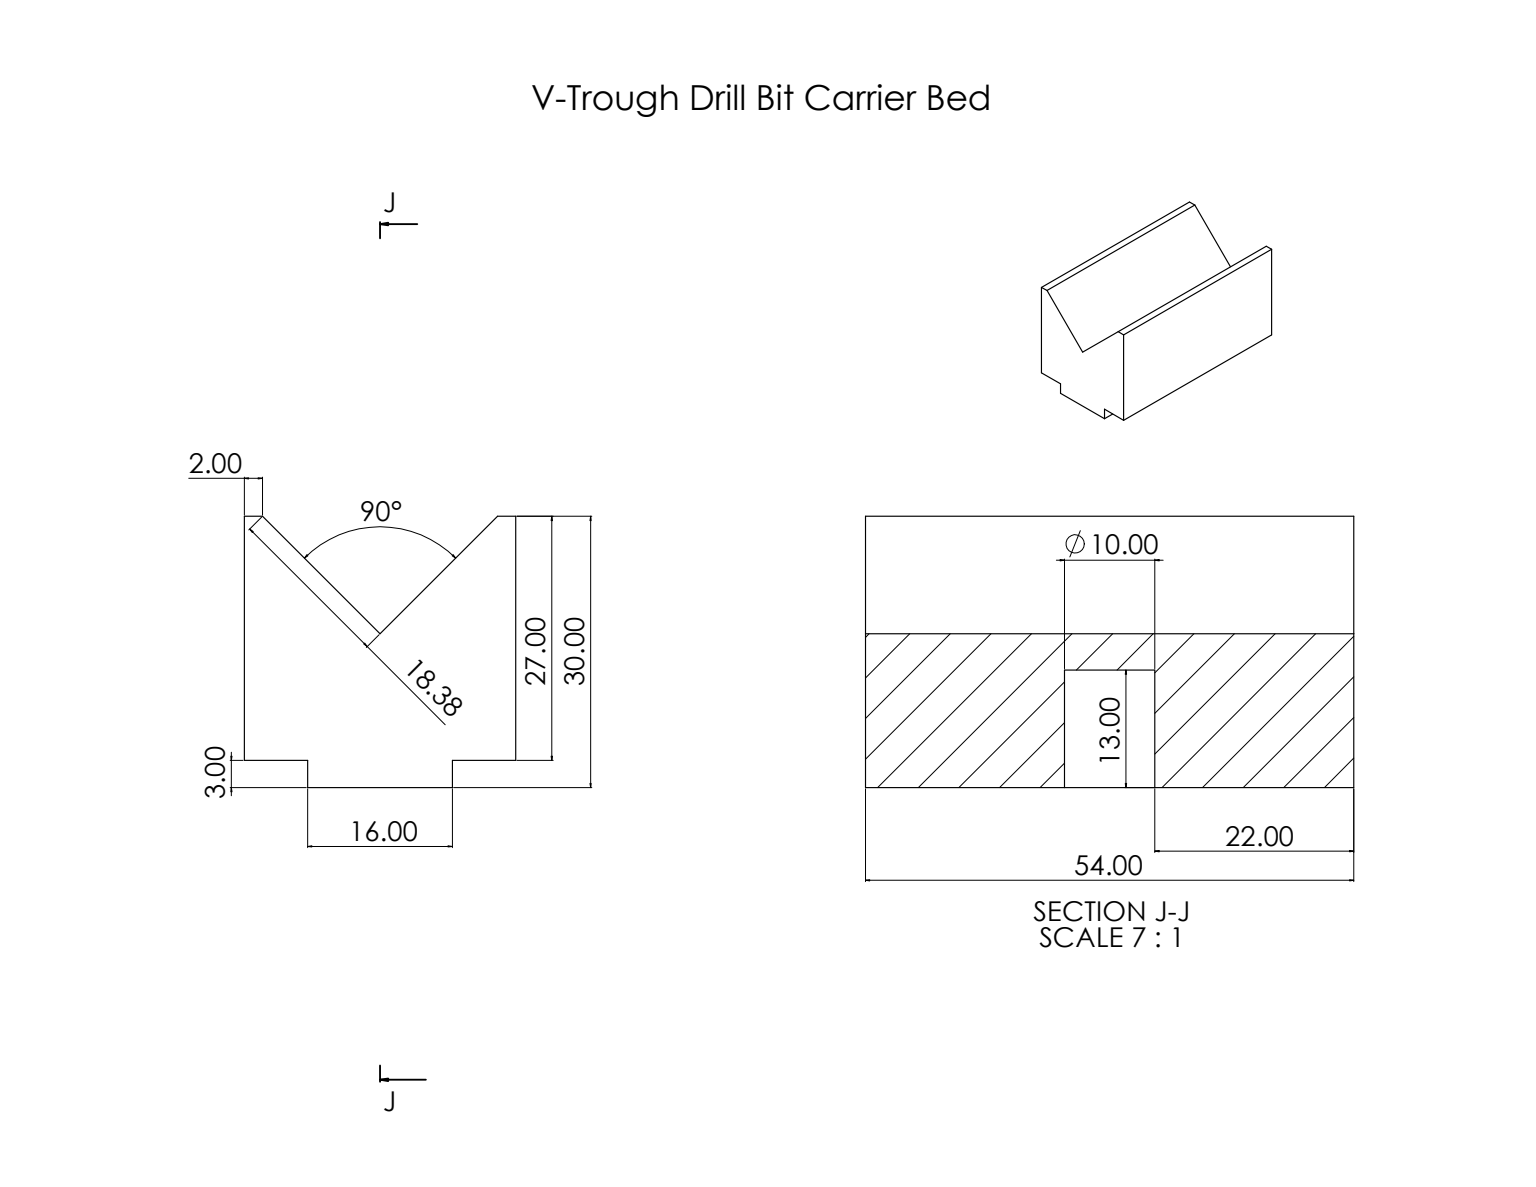
ISO-10303-21;
HEADER;
FILE_DESCRIPTION (('STEP AP214'),
    '1' );
FILE_NAME ('V-Trough Drill Bit Carrier Bed.step',
    '2026-10-26T22:46:44',
    ( '' ),
    ( '' ),
    'SwSTEP 2.0',
    'SolidWorks 2025',
    '' );
FILE_SCHEMA (( 'AUTOMOTIVE_DESIGN' ));
ENDSEC;

DATA;
#6=ORIENTED_EDGE ( 'NONE', *, *, #8024, .T. ) ;
#20=LINE ( 'NONE', #125, #6600 ) ;
#91=EDGE_CURVE ( 'NONE', #17637, #19670, #15056, .T. ) ;
#99=ORIENTED_EDGE ( 'NONE', *, *, #8969, .F. ) ;
#125=CARTESIAN_POINT ( 'NONE',  ( 74.11964624731606932, 223.5773763115391262, -13.99999999999998757 ) ) ;
#138=VECTOR ( 'NONE', #4761, 1000.000000000000114 ) ;
#144=ORIENTED_EDGE ( 'NONE', *, *, #2804, .F. ) ;
#147=CARTESIAN_POINT ( 'NONE',  ( 59.39721438298058587, 215.0773763115390125, -5.999999999999973355 ) ) ;
#214=ORIENTED_EDGE ( 'NONE', *, *, #1106, .F. ) ;
#252=ORIENTED_EDGE ( 'NONE', *, *, #4604, .T. ) ;
#276=DIRECTION ( 'NONE',  ( 0.000000000000000000, 0.000000000000000000, -1.000000000000000000 ) ) ;
#283=DIRECTION ( 'NONE',  ( -0.8660254037844370423, -0.5000000000000027756, 0.000000000000000000 ) ) ;
#292=ORIENTED_EDGE ( 'NONE', *, *, #18582, .T. ) ;
#382=AXIS2_PLACEMENT_3D ( 'NONE', #19245, #4714, #11186 ) ;
#397=DIRECTION ( 'NONE',  ( -0.8660254037844360431, -0.5000000000000046629, 0.000000000000000000 ) ) ;
#416=LINE ( 'NONE', #6862, #13294 ) ;
#757=DIRECTION ( 'NONE',  ( -3.965082230804136925E-15, -7.930164461608273850E-15, 1.000000000000000000 ) ) ;
#780=CARTESIAN_POINT ( 'NONE',  ( 61.99529059433385925, 216.5773763115390125, -5.999999999999973355 ) ) ;
#823=EDGE_LOOP ( 'NONE', ( #9472, #292, #20590, #17271 ) ) ;
#881=PLANE ( 'NONE',  #5818 ) ;
#968=EDGE_CURVE ( 'NONE', #15204, #2259, #12531, .T. ) ;
#983=CIRCLE ( 'NONE', #5694, 5.000000000000005329 ) ;
#986=PRODUCT_DEFINITION_FORMATION_WITH_SPECIFIED_SOURCE ( 'ANY', '', #7367, .NOT_KNOWN. ) ;
#1094=( GEOMETRIC_REPRESENTATION_CONTEXT ( 3 ) GLOBAL_UNCERTAINTY_ASSIGNED_CONTEXT ( ( #5747 ) ) GLOBAL_UNIT_ASSIGNED_CONTEXT ( ( #17535, #19424, #17849 ) ) REPRESENTATION_CONTEXT ( 'NONE', 'WORKASPACE' ) );
#1106=EDGE_CURVE ( 'NONE', #19041, #17375, #6452, .T. ) ;
#1124=LINE ( 'NONE', #12466, #4797 ) ;
#1130=DIRECTION ( 'NONE',  ( -0.8660254037844370423, -0.5000000000000027756, -0.000000000000000000 ) ) ;
#1156=VECTOR ( 'NONE', #15622, 1000.000000000000000 ) ;
#1183=ORIENTED_EDGE ( 'NONE', *, *, #12632, .F. ) ;
#1214=VECTOR ( 'NONE', #5254, 1000.000000000000227 ) ;
#1274=DIRECTION ( 'NONE',  ( 0.000000000000000000, 0.000000000000000000, 1.000000000000000000 ) ) ;
#1588=VERTEX_POINT ( 'NONE', #19080 ) ;
#1594=VERTEX_POINT ( 'NONE', #18972 ) ;
#1643=ORIENTED_EDGE ( 'NONE', *, *, #12632, .T. ) ;
#1738=DIRECTION ( 'NONE',  ( -3.965082230804136925E-15, -7.930164461608273850E-15, 1.000000000000000000 ) ) ;
#1796=SHAPE_REPRESENTATION ( 'V-Trough Drill Bit Carrier Bed', ( #18233 ), #14188 ) ;
#1868=ORIENTED_EDGE ( 'NONE', *, *, #14937, .T. ) ;
#1885=DIRECTION ( 'NONE',  ( 0.8660254037844348218, 0.5000000000000064393, 0.000000000000000000 ) ) ;
#1887=DIRECTION ( 'NONE',  ( -0.5000000000000045519, 0.8660254037844360431, 0.000000000000000000 ) ) ;
#1915=EDGE_LOOP ( 'NONE', ( #17865, #19620, #6, #15097 ) ) ;
#1955=AXIS2_PLACEMENT_3D ( 'NONE', #14799, #5313, #4911 ) ;
#1958=VERTEX_POINT ( 'NONE', #20807 ) ;
#2005=ADVANCED_FACE ( 'NONE', ( #9459 ), #4907, .F. ) ;
#2016=VERTEX_POINT ( 'NONE', #6380 ) ;
#2098=VERTEX_POINT ( 'NONE', #9771 ) ;
#2104=EDGE_LOOP ( 'NONE', ( #1183, #10709, #4662, #6785 ) ) ;
#2110=EDGE_CURVE ( 'NONE', #2016, #10851, #18262, .T. ) ;
#2208=DIRECTION ( 'NONE',  ( -0.5000000000000045519, 0.8660254037844360431, 0.000000000000000000 ) ) ;
#2259=VERTEX_POINT ( 'NONE', #4046 ) ;
#2305=PLANE ( 'NONE',  #19993 ) ;
#2322=FACE_OUTER_BOUND ( 'NONE', #2755, .T. ) ;
#2325=VERTEX_POINT ( 'NONE', #7748 ) ;
#2343=CARTESIAN_POINT ( 'NONE',  ( 74.11964624731606932, 223.5773763115391262, -13.99999999999998757 ) ) ;
#2376=VECTOR ( 'NONE', #276, 1000.000000000000000 ) ;
#2395=LINE ( 'NONE', #5765, #14247 ) ;
#2423=ADVANCED_FACE ( 'NONE', ( #9545 ), #20784, .T. ) ;
#2503=AXIS2_PLACEMENT_3D ( 'NONE', #12544, #7650, #2794 ) ;
#2539=VERTEX_POINT ( 'NONE', #11222 ) ;
#2566=EDGE_CURVE ( 'NONE', #19041, #1588, #11424, .T. ) ;
#2697=DIRECTION ( 'NONE',  ( -0.5000000000000027756, 0.8660254037844370423, -4.885182764539217401E-15 ) ) ;
#2755=EDGE_LOOP ( 'NONE', ( #15288, #4387, #20400, #14266 ) ) ;
#2772=ADVANCED_FACE ( 'NONE', ( #10120 ), #2305, .T. ) ;
#2773=VERTEX_POINT ( 'NONE', #6735 ) ;
#2776=ORIENTED_EDGE ( 'NONE', *, *, #4882, .F. ) ;
#2794=DIRECTION ( 'NONE',  ( -0.7559289460184535070, 0.000000000000000000, -0.6546536707079781969 ) ) ;
#2804=EDGE_CURVE ( 'NONE', #9345, #7191, #6784, .T. ) ;
#2819=DIRECTION ( 'NONE',  ( 0.8660254037844370423, 0.5000000000000027756, 0.000000000000000000 ) ) ;
#2887=DIRECTION ( 'NONE',  ( -0.8660254037844362651, -0.5000000000000045519, 5.976026924694053325E-17 ) ) ;
#2949=VERTEX_POINT ( 'NONE', #17764 ) ;
#2995=DIRECTION ( 'NONE',  ( 0.5000000000000045519, -0.8660254037844360431, 0.000000000000000000 ) ) ;
#3089=EDGE_CURVE ( 'NONE', #5258, #2325, #16478, .T. ) ;
#3121=DIRECTION ( 'NONE',  ( -0.8660254037844360431, -0.5000000000000044409, 5.976026924694052093E-17 ) ) ;
#3123=CARTESIAN_POINT ( 'NONE',  ( 61.99529059433388767, 216.5773763115390693, -28.99999999999998934 ) ) ;
#3124=ORIENTED_EDGE ( 'NONE', *, *, #968, .T. ) ;
#3158=ORIENTED_EDGE ( 'NONE', *, *, #14937, .F. ) ;
#3194=DIRECTION ( 'NONE',  ( -0.8660254037844360431, -0.5000000000000045519, -7.398944170774820286E-15 ) ) ;
#3316=ORIENTED_EDGE ( 'NONE', *, *, #3433, .F. ) ;
#3331=MANIFOLD_SOLID_BREP ( 'Cut-Extrude5', #10659 ) ;
#3424=FACE_OUTER_BOUND ( 'NONE', #20462, .T. ) ;
#3426=EDGE_CURVE ( 'NONE', #17375, #2098, #9056, .T. ) ;
#3433=EDGE_CURVE ( 'NONE', #18964, #2773, #2395, .T. ) ;
#3547=ORIENTED_EDGE ( 'NONE', *, *, #13844, .T. ) ;
#3597=CARTESIAN_POINT ( 'NONE',  ( 58.37797649651341203, 276.8427481158987007, -26.99999999999999289 ) ) ;
#3605=CARTESIAN_POINT ( 'NONE',  ( 61.99529059433388767, 216.5773763115390693, 1.000000000000017097 ) ) ;
#3728=CARTESIAN_POINT ( 'NONE',  ( 85.37797649651368204, 230.0773763115391262, -26.99999999999999289 ) ) ;
#3788=CARTESIAN_POINT ( 'NONE',  ( 85.37797649651368204, 230.0773763115391262, -28.99999999999998934 ) ) ;
#3847=VECTOR ( 'NONE', #6152, 1000.000000000000114 ) ;
#3889=LINE ( 'NONE', #10341, #13471 ) ;
#3959=DIRECTION ( 'NONE',  ( -0.8660254037844370423, -0.5000000000000027756, 0.000000000000000000 ) ) ;
#3988=CARTESIAN_POINT ( 'NONE',  ( 85.37797649651368204, 230.0773763115391262, -28.99999999999998934 ) ) ;
#4046=CARTESIAN_POINT ( 'NONE',  ( 58.37797649651341203, 276.8427481158987007, -0.9999999999999826805 ) ) ;
#4155=CARTESIAN_POINT ( 'NONE',  ( 58.37797649651341203, 276.8427481158987007, 1.000000000000017097 ) ) ;
#4215=CARTESIAN_POINT ( 'NONE',  ( 85.37797649651368204, 230.0773763115391262, -26.99999999999999289 ) ) ;
#4282=EDGE_LOOP ( 'NONE', ( #144, #17540 ) ) ;
#4380=LINE ( 'NONE', #18697, #12901 ) ;
#4387=ORIENTED_EDGE ( 'NONE', *, *, #7070, .F. ) ;
#4476=LINE ( 'NONE', #18685, #13839 ) ;
#4604=EDGE_CURVE ( 'NONE', #4855, #18774, #12621, .T. ) ;
#4642=ORIENTED_EDGE ( 'NONE', *, *, #2566, .T. ) ;
#4662=ORIENTED_EDGE ( 'NONE', *, *, #11730, .T. ) ;
#4677=CARTESIAN_POINT ( 'NONE',  ( 61.99529059433388767, 216.5773763115390693, -28.99999999999998934 ) ) ;
#4714=DIRECTION ( 'NONE',  ( -0.8660254037844360431, -0.5000000000000045519, 0.000000000000000000 ) ) ;
#4754=CARTESIAN_POINT ( 'NONE',  ( 34.99529059433359635, 263.3427481158985870, -22.00000000000000355 ) ) ;
#4761=DIRECTION ( 'NONE',  ( 0.8660254037844348218, 0.5000000000000064393, 0.000000000000000000 ) ) ;
#4787=VECTOR ( 'NONE', #16383, 1000.000000000000000 ) ;
#4797=VECTOR ( 'NONE', #2819, 1000.000000000000114 ) ;
#4814=CYLINDRICAL_SURFACE ( 'NONE', #1955, 5.000000000000005329 ) ;
#4855=VERTEX_POINT ( 'NONE', #12972 ) ;
#4882=EDGE_CURVE ( 'NONE', #2539, #19041, #13377, .T. ) ;
#4907=CYLINDRICAL_SURFACE ( 'NONE', #13362, 5.000000000000005329 ) ;
#4911=DIRECTION ( 'NONE',  ( 0.5000000000000041078, -0.8660254037844363761, 0.000000000000000000 ) ) ;
#5011=DIRECTION ( 'NONE',  ( -0.5000000000000045519, 0.8660254037844360431, 0.000000000000000000 ) ) ;
#5026=CARTESIAN_POINT ( 'NONE',  ( 32.39721438298032297, 261.8427481158985870, -22.00000000000000355 ) ) ;
#5056=DIRECTION ( 'NONE',  ( 0.8660254037844360431, 0.5000000000000045519, -0.000000000000000000 ) ) ;
#5062=DIRECTION ( 'NONE',  ( 0.5000000000000044409, -0.8660254037844361541, 0.000000000000000000 ) ) ;
#5077=EDGE_LOOP ( 'NONE', ( #10295, #3158, #12362, #12866 ) ) ;
#5087=CARTESIAN_POINT ( 'NONE',  ( 43.39721438298041534, 242.7901892326410120, -13.99999999999998046 ) ) ;
#5168=VECTOR ( 'NONE', #757, 1000.000000000000000 ) ;
#5171=ORIENTED_EDGE ( 'NONE', *, *, #9282, .F. ) ;
#5254=DIRECTION ( 'NONE',  ( -0.6123724356957914727, -0.3535533905932749521, -0.7071067811865495711 ) ) ;
#5258=VERTEX_POINT ( 'NONE', #20026 ) ;
#5313=DIRECTION ( 'NONE',  ( -0.8660254037844360431, -0.5000000000000044409, 5.976026924694052093E-17 ) ) ;
#5370=DIRECTION ( 'NONE',  ( 1.000000000000000000, 0.000000000000000000, -0.000000000000000000 ) ) ;
#5433=( LENGTH_UNIT ( ) NAMED_UNIT ( * ) SI_UNIT ( .MILLI., .METRE. ) );
#5452=DIRECTION ( 'NONE',  ( -0.000000000000000000, -0.000000000000000000, -1.000000000000000000 ) ) ;
#5538=PLANE ( 'NONE',  #16869 ) ;
#5564=EDGE_CURVE ( 'NONE', #2098, #5258, #8016, .T. ) ;
#5566=DIRECTION ( 'NONE',  ( -0.8660254037844360431, -0.5000000000000045519, 7.398944170774818708E-15 ) ) ;
#5638=FACE_OUTER_BOUND ( 'NONE', #20459, .T. ) ;
#5660=DIRECTION ( 'NONE',  ( -0.8660254037844370423, -0.5000000000000027756, -0.000000000000000000 ) ) ;
#5667=CARTESIAN_POINT ( 'NONE',  ( 57.15554463217811332, 244.9600622137188850, -13.99999999999998046 ) ) ;
#5683=CARTESIAN_POINT ( 'NONE',  ( 61.99529059433388767, 216.5773763115390693, 1.000000000000017097 ) ) ;
#5694=AXIS2_PLACEMENT_3D ( 'NONE', #17303, #2887, #5938 ) ;
#5735=DIRECTION ( 'NONE',  ( 0.6123724356957914727, 0.3535533905932749521, -0.7071067811865495711 ) ) ;
#5747=UNCERTAINTY_MEASURE_WITH_UNIT (LENGTH_MEASURE( 1.000000000000000082E-05 ), #17535, 'distance_accuracy_value', 'NONE');
#5764=EDGE_CURVE ( 'NONE', #2325, #15204, #1124, .T. ) ;
#5765=CARTESIAN_POINT ( 'NONE',  ( 61.99529059433388767, 216.5773763115390693, -28.99999999999998934 ) ) ;
#5778=CARTESIAN_POINT ( 'NONE',  ( 45.89721438298043665, 238.4600622137188282, -13.99999999999998046 ) ) ;
#5811=EDGE_LOOP ( 'NONE', ( #20591, #9670, #12240, #1868 ) ) ;
#5818=AXIS2_PLACEMENT_3D ( 'NONE', #15325, #13818, #20068 ) ;
#5890=PLANE ( 'NONE',  #16334 ) ;
#5907=ADVANCED_FACE ( 'NONE', ( #11803 ), #881, .T. ) ;
#5935=PRODUCT_CONTEXT ( 'NONE', #15314, 'mechanical' ) ;
#5938=DIRECTION ( 'NONE',  ( 0.5000000000000041078, -0.8660254037844363761, 0.000000000000000000 ) ) ;
#5981=FACE_BOUND ( 'NONE', #4282, .T. ) ;
#6003=CARTESIAN_POINT ( 'NONE',  ( 85.37797649651368204, 230.0773763115391262, -28.99999999999998934 ) ) ;
#6083=PLANE ( 'NONE',  #382 ) ;
#6111=ORIENTED_EDGE ( 'NONE', *, *, #7734, .F. ) ;
#6152=DIRECTION ( 'NONE',  ( -0.5000000000000045519, 0.8660254037844360431, 0.000000000000000000 ) ) ;
#6350=VECTOR ( 'NONE', #8825, 1000.000000000000114 ) ;
#6380=CARTESIAN_POINT ( 'NONE',  ( 85.37797649651368204, 230.0773763115391262, -26.99999999999999289 ) ) ;
#6382=DIRECTION ( 'NONE',  ( 1.000000000000000000, 0.000000000000000000, -0.000000000000000000 ) ) ;
#6410=CARTESIAN_POINT ( 'NONE',  ( 85.37797649651368204, 230.0773763115391262, 1.000000000000017097 ) ) ;
#6452=LINE ( 'NONE', #17821, #3847 ) ;
#6458=CARTESIAN_POINT ( 'NONE',  ( 59.65554463217813463, 240.6299351947967011, -13.99999999999998046 ) ) ;
#6512=LINE ( 'NONE', #6616, #13600 ) ;
#6521=DIRECTION ( 'NONE',  ( 0.5000000000000041078, -0.8660254037844363761, 0.000000000000000000 ) ) ;
#6559=DIRECTION ( 'NONE',  ( -0.5000000000000045519, 0.8660254037844360431, 0.000000000000000000 ) ) ;
#6564=DIRECTION ( 'NONE',  ( -0.8660254037844361541, -0.5000000000000044409, 5.976026924694052093E-17 ) ) ;
#6600=VECTOR ( 'NONE', #6559, 1000.000000000000114 ) ;
#6616=CARTESIAN_POINT ( 'NONE',  ( 85.37797649651368204, 230.0773763115391262, -0.9999999999999826805 ) ) ;
#6636=AXIS2_PLACEMENT_3D ( 'NONE', #8437, #11527, #1887 ) ;
#6644=PLANE ( 'NONE',  #13908 ) ;
#6655=ORIENTED_EDGE ( 'NONE', *, *, #2804, .T. ) ;
#6712=ORIENTED_EDGE ( 'NONE', *, *, #3426, .T. ) ;
#6735=CARTESIAN_POINT ( 'NONE',  ( 61.99529059433388767, 216.5773763115390693, -28.99999999999998934 ) ) ;
#6784=CIRCLE ( 'NONE', #17992, 5.000000000000005329 ) ;
#6785=ORIENTED_EDGE ( 'NONE', *, *, #17239, .T. ) ;
#6862=CARTESIAN_POINT ( 'NONE',  ( 61.99529059433385925, 216.5773763115390125, -5.999999999999973355 ) ) ;
#6969=DIRECTION ( 'NONE',  ( 0.000000000000000000, 0.000000000000000000, -1.000000000000000000 ) ) ;
#6987=VECTOR ( 'NONE', #8149, 1000.000000000000227 ) ;
#6993=LINE ( 'NONE', #8591, #8467 ) ;
#7058=CARTESIAN_POINT ( 'NONE',  ( 32.39721438298032297, 261.8427481158985870, -5.999999999999973355 ) ) ;
#7070=EDGE_CURVE ( 'NONE', #1958, #2325, #6993, .T. ) ;
#7191=VERTEX_POINT ( 'NONE', #5087 ) ;
#7276=PLANE ( 'NONE',  #18043 ) ;
#7367=PRODUCT ( 'V-Trough Drill Bit Carrier Bed', 'V-Trough Drill Bit Carrier Bed', '', ( #5935 ) ) ;
#7396=CARTESIAN_POINT ( 'NONE',  ( 85.37797649651368204, 230.0773763115391262, 1.000000000000017097 ) ) ;
#7569=ADVANCED_FACE ( 'NONE', ( #10134 ), #6644, .T. ) ;
#7604=LINE ( 'NONE', #6003, #17983 ) ;
#7618=ADVANCED_FACE ( 'NONE', ( #2322 ), #7276, .T. ) ;
#7650=DIRECTION ( 'NONE',  ( 0.6123724356957944703, 0.3535533905932780607, -0.7071067811865454633 ) ) ;
#7734=EDGE_CURVE ( 'NONE', #11978, #5258, #10775, .T. ) ;
#7739=ORIENTED_EDGE ( 'NONE', *, *, #17717, .T. ) ;
#7748=CARTESIAN_POINT ( 'NONE',  ( 34.99529059433362477, 263.3427481158986438, 1.000000000000017097 ) ) ;
#7815=ADVANCED_BREP_SHAPE_REPRESENTATION ( '', ( #3331, #18233 ), #14188 ) ;
#7887=ORIENTED_EDGE ( 'NONE', *, *, #8024, .F. ) ;
#7913=ORIENTED_EDGE ( 'NONE', *, *, #10333, .F. ) ;
#7922=EDGE_LOOP ( 'NONE', ( #11863, #6111, #10020, #18675 ) ) ;
#7955=LINE ( 'NONE', #6458, #10564 ) ;
#8016=LINE ( 'NONE', #7058, #8477 ) ;
#8024=EDGE_CURVE ( 'NONE', #16809, #17637, #14825, .T. ) ;
#8111=CARTESIAN_POINT ( 'NONE',  ( 45.89721438298043665, 238.4600622137188282, -13.99999999999998046 ) ) ;
#8125=EDGE_CURVE ( 'NONE', #2949, #15199, #8853, .T. ) ;
#8149=DIRECTION ( 'NONE',  ( 0.6123724356957914727, 0.3535533905932749521, -0.7071067811865495711 ) ) ;
#8220=FACE_OUTER_BOUND ( 'NONE', #20198, .T. ) ;
#8272=CARTESIAN_POINT ( 'NONE',  ( 61.99529059433385925, 216.5773763115390125, -22.00000000000000355 ) ) ;
#8287=PLANE ( 'NONE',  #8526 ) ;
#8291=LINE ( 'NONE', #11599, #11107 ) ;
#8351=CARTESIAN_POINT ( 'NONE',  ( 61.99529059433385925, 216.5773763115390125, -22.00000000000000355 ) ) ;
#8437=CARTESIAN_POINT ( 'NONE',  ( 85.37797649651368204, 230.0773763115391262, 1.000000000000017097 ) ) ;
#8452=DIRECTION ( 'NONE',  ( -1.000000000000000000, 0.000000000000000000, 0.000000000000000000 ) ) ;
#8467=VECTOR ( 'NONE', #15089, 1000.000000000000114 ) ;
#8477=VECTOR ( 'NONE', #1885, 1000.000000000000114 ) ;
#8526=AXIS2_PLACEMENT_3D ( 'NONE', #147, #14797, #6382 ) ;
#8591=CARTESIAN_POINT ( 'NONE',  ( 61.99529059433388767, 216.5773763115390693, 1.000000000000017097 ) ) ;
#8734=EDGE_CURVE ( 'NONE', #19670, #2016, #4380, .T. ) ;
#8825=DIRECTION ( 'NONE',  ( -0.8660254037844348218, -0.5000000000000064393, 0.000000000000000000 ) ) ;
#8826=ORIENTED_EDGE ( 'NONE', *, *, #19765, .F. ) ;
#8853=LINE ( 'NONE', #18512, #13885 ) ;
#8880=DIRECTION ( 'NONE',  ( 0.000000000000000000, -0.000000000000000000, 1.000000000000000000 ) ) ;
#8969=EDGE_CURVE ( 'NONE', #18964, #2949, #7604, .T. ) ;
#9056=LINE ( 'NONE', #9157, #10125 ) ;
#9117=EDGE_CURVE ( 'NONE', #7191, #9345, #12571, .T. ) ;
#9152=ADVANCED_FACE ( 'NONE', ( #8220 ), #16405, .F. ) ;
#9157=CARTESIAN_POINT ( 'NONE',  ( 32.39721438298032297, 261.8427481158985870, -22.00000000000000355 ) ) ;
#9282=EDGE_CURVE ( 'NONE', #2016, #18964, #15151, .T. ) ;
#9301=LINE ( 'NONE', #14222, #15228 ) ;
#9316=ORIENTED_EDGE ( 'NONE', *, *, #8969, .T. ) ;
#9320=SHAPE_DEFINITION_REPRESENTATION ( #17040, #1796 ) ;
#9345=VERTEX_POINT ( 'NONE', #12473 ) ;
#9441=ADVANCED_FACE ( 'NONE', ( #5981, #11080 ), #6083, .T. ) ;
#9459=FACE_OUTER_BOUND ( 'NONE', #823, .T. ) ;
#9472=ORIENTED_EDGE ( 'NONE', *, *, #4604, .F. ) ;
#9524=LINE ( 'NONE', #11337, #138 ) ;
#9545=FACE_OUTER_BOUND ( 'NONE', #2104, .T. ) ;
#9670=ORIENTED_EDGE ( 'NONE', *, *, #10637, .F. ) ;
#9739=ORIENTED_EDGE ( 'NONE', *, *, #5564, .T. ) ;
#9771=CARTESIAN_POINT ( 'NONE',  ( 32.39721438298032297, 261.8427481158985870, -5.999999999999973355 ) ) ;
#9808=DIRECTION ( 'NONE',  ( -0.5000000000000027756, 0.8660254037844370423, -4.885182764539217401E-15 ) ) ;
#9838=LINE ( 'NONE', #3597, #6987 ) ;
#10020=ORIENTED_EDGE ( 'NONE', *, *, #10333, .T. ) ;
#10098=( NAMED_UNIT ( * ) PLANE_ANGLE_UNIT ( ) SI_UNIT ( $, .RADIAN. ) );
#10120=FACE_OUTER_BOUND ( 'NONE', #7922, .T. ) ;
#10125=VECTOR ( 'NONE', #16914, 1000.000000000000000 ) ;
#10129=FACE_OUTER_BOUND ( 'NONE', #13772, .T. ) ;
#10134=FACE_OUTER_BOUND ( 'NONE', #11173, .T. ) ;
#10155=AXIS2_PLACEMENT_3D ( 'NONE', #17898, #9808, #283 ) ;
#10226=DIRECTION ( 'NONE',  ( -0.8660254037844362651, -0.5000000000000045519, 5.976026924694053325E-17 ) ) ;
#10238=CARTESIAN_POINT ( 'NONE',  ( 85.37797649651368204, 230.0773763115391262, -28.99999999999998934 ) ) ;
#10247=VERTEX_POINT ( 'NONE', #4754 ) ;
#10294=LINE ( 'NONE', #15425, #6350 ) ;
#10295=ORIENTED_EDGE ( 'NONE', *, *, #16540, .F. ) ;
#10333=EDGE_CURVE ( 'NONE', #11978, #1958, #416, .T. ) ;
#10341=CARTESIAN_POINT ( 'NONE',  ( 61.99529059433385925, 216.5773763115390125, -22.00000000000000355 ) ) ;
#10366=LINE ( 'NONE', #15396, #19904 ) ;
#10448=AXIS2_PLACEMENT_3D ( 'NONE', #3788, #5056, #2208 ) ;
#10540=ADVANCED_FACE ( 'NONE', ( #15991 ), #5890, .T. ) ;
#10564=VECTOR ( 'NONE', #6564, 1000.000000000000227 ) ;
#10612=DIRECTION ( 'NONE',  ( -0.5000000000000045519, 0.8660254037844360431, 0.000000000000000000 ) ) ;
#10637=EDGE_CURVE ( 'NONE', #17637, #2259, #6512, .T. ) ;
#10659=CLOSED_SHELL ( 'NONE', ( #2005, #2772, #11755, #9441, #14116, #2423, #5907, #18948, #10540, #13296, #15791, #7618, #9152, #17917, #20296, #7569 ) ) ;
#10709=ORIENTED_EDGE ( 'NONE', *, *, #17717, .F. ) ;
#10775=LINE ( 'NONE', #12701, #20646 ) ;
#10851=VERTEX_POINT ( 'NONE', #15867 ) ;
#10864=ORIENTED_EDGE ( 'NONE', *, *, #16540, .T. ) ;
#10959=ORIENTED_EDGE ( 'NONE', *, *, #3089, .T. ) ;
#11080=FACE_OUTER_BOUND ( 'NONE', #17131, .T. ) ;
#11107=VECTOR ( 'NONE', #5011, 1000.000000000000114 ) ;
#11114=DIRECTION ( 'NONE',  ( 0.000000000000000000, 0.000000000000000000, 1.000000000000000000 ) ) ;
#11173=EDGE_LOOP ( 'NONE', ( #18387, #252 ) ) ;
#11178=FACE_OUTER_BOUND ( 'NONE', #18616, .T. ) ;
#11186=DIRECTION ( 'NONE',  ( 0.5000000000000045519, -0.8660254037844360431, 0.000000000000000000 ) ) ;
#11222=CARTESIAN_POINT ( 'NONE',  ( 61.99529059433385925, 216.5773763115390125, -22.00000000000000355 ) ) ;
#11236=DIRECTION ( 'NONE',  ( 3.965082230804136136E-15, 7.930164461608272272E-15, 1.000000000000000000 ) ) ;
#11307=DIRECTION ( 'NONE',  ( -0.5000000000000045519, 0.8660254037844360431, 0.000000000000000000 ) ) ;
#11337=CARTESIAN_POINT ( 'NONE',  ( 59.39721438298058587, 215.0773763115390125, -5.999999999999973355 ) ) ;
#11392=ORIENTED_EDGE ( 'NONE', *, *, #9282, .T. ) ;
#11424=LINE ( 'NONE', #17903, #13925 ) ;
#11483=LINE ( 'NONE', #3123, #19361 ) ;
#11527=DIRECTION ( 'NONE',  ( 0.8660254037844360431, 0.5000000000000045519, 0.000000000000000000 ) ) ;
#11544=ORIENTED_EDGE ( 'NONE', *, *, #7734, .T. ) ;
#11599=CARTESIAN_POINT ( 'NONE',  ( 59.39721438298058587, 215.0773763115390125, -5.999999999999973355 ) ) ;
#11730=EDGE_CURVE ( 'NONE', #2773, #2539, #11483, .T. ) ;
#11755=ADVANCED_FACE ( 'NONE', ( #3424 ), #8287, .T. ) ;
#11803=FACE_OUTER_BOUND ( 'NONE', #12053, .T. ) ;
#11815=CARTESIAN_POINT ( 'NONE',  ( 34.99529059433359635, 263.3427481158985870, -5.999999999999973355 ) ) ;
#11862=FACE_OUTER_BOUND ( 'NONE', #15817, .T. ) ;
#11863=ORIENTED_EDGE ( 'NONE', *, *, #3089, .F. ) ;
#11923=STYLED_ITEM('',(#20974),#3331);
#11978=VERTEX_POINT ( 'NONE', #780 ) ;
#12053=EDGE_LOOP ( 'NONE', ( #16727, #99, #18551, #7739 ) ) ;
#12059=DIRECTION ( 'NONE',  ( 0.5000000000000045519, -0.8660254037844360431, 0.000000000000000000 ) ) ;
#12064=AXIS2_PLACEMENT_3D ( 'NONE', #8351, #6969, #8452 ) ;
#12138=SHAPE_REPRESENTATION_RELATIONSHIP ( 'NONE' , 'NONE' ,  #1796, #7815 ) ;
#12190=VECTOR ( 'NONE', #14782, 1000.000000000000114 ) ;
#12217=CARTESIAN_POINT ( 'NONE',  ( 58.37797649651341203, 276.8427481158987007, 1.000000000000017097 ) ) ;
#12240=ORIENTED_EDGE ( 'NONE', *, *, #91, .T. ) ;
#12286=EDGE_CURVE ( 'NONE', #18774, #9345, #7955, .T. ) ;
#12298=ORIENTED_EDGE ( 'NONE', *, *, #3426, .F. ) ;
#12311=DIRECTION ( 'NONE',  ( -0.6123724356957914727, -0.3535533905932749521, -0.7071067811865495711 ) ) ;
#12362=ORIENTED_EDGE ( 'NONE', *, *, #8734, .T. ) ;
#12466=CARTESIAN_POINT ( 'NONE',  ( 34.99529059433362477, 263.3427481158986438, 1.000000000000017097 ) ) ;
#12473=CARTESIAN_POINT ( 'NONE',  ( 48.39721438298045797, 234.1299351947966443, -13.99999999999998046 ) ) ;
#12479=DIRECTION ( 'NONE',  ( 0.5000000000000041078, -0.8660254037844363761, 0.000000000000000000 ) ) ;
#12505=VECTOR ( 'NONE', #13892, 1000.000000000000227 ) ;
#12531=LINE ( 'NONE', #12217, #1156 ) ;
#12544=CARTESIAN_POINT ( 'NONE',  ( 85.37797649651368204, 230.0773763115391262, -0.9999999999999826805 ) ) ;
#12571=CIRCLE ( 'NONE', #16967, 5.000000000000005329 ) ;
#12621=CIRCLE ( 'NONE', #16242, 5.000000000000005329 ) ;
#12632=EDGE_CURVE ( 'NONE', #15199, #10247, #18978, .T. ) ;
#12701=CARTESIAN_POINT ( 'NONE',  ( 61.99529059433385925, 216.5773763115390125, -5.999999999999973355 ) ) ;
#12866=ORIENTED_EDGE ( 'NONE', *, *, #2110, .T. ) ;
#12880=PRODUCT_DEFINITION ( 'UNKNOWN', '', #986, #20391 ) ;
#12901=VECTOR ( 'NONE', #5735, 1000.000000000000227 ) ;
#12925=PLANE ( 'NONE',  #6636 ) ;
#12972=CARTESIAN_POINT ( 'NONE',  ( 54.65554463217808490, 249.2901892326410689, -13.99999999999998046 ) ) ;
#13140=CARTESIAN_POINT ( 'NONE',  ( 57.15554463217811332, 244.9600622137188850, -13.99999999999998046 ) ) ;
#13294=VECTOR ( 'NONE', #11236, 1000.000000000000000 ) ;
#13296=ADVANCED_FACE ( 'NONE', ( #15736 ), #17521, .T. ) ;
#13317=ORIENTED_EDGE ( 'NONE', *, *, #18738, .T. ) ;
#13362=AXIS2_PLACEMENT_3D ( 'NONE', #14584, #3121, #15959 ) ;
#13377=LINE ( 'NONE', #8272, #12190 ) ;
#13471=VECTOR ( 'NONE', #15262, 1000.000000000000114 ) ;
#13600=VECTOR ( 'NONE', #11307, 1000.000000000000114 ) ;
#13772=EDGE_LOOP ( 'NONE', ( #18422, #16263, #11392, #9316 ) ) ;
#13818=DIRECTION ( 'NONE',  ( 0.000000000000000000, 0.000000000000000000, -1.000000000000000000 ) ) ;
#13839=VECTOR ( 'NONE', #10612, 1000.000000000000114 ) ;
#13844=EDGE_CURVE ( 'NONE', #1588, #11978, #9524, .T. ) ;
#13869=DIRECTION ( 'NONE',  ( 0.6123724356957944703, 0.3535533905932780607, 0.7071067811865454633 ) ) ;
#13885=VECTOR ( 'NONE', #5660, 1000.000000000000114 ) ;
#13892=DIRECTION ( 'NONE',  ( -0.8660254037844361541, -0.5000000000000044409, 5.976026924694052093E-17 ) ) ;
#13908=AXIS2_PLACEMENT_3D ( 'NONE', #13140, #19584, #5062 ) ;
#13925=VECTOR ( 'NONE', #11114, 1000.000000000000000 ) ;
#14052=UNCERTAINTY_MEASURE_WITH_UNIT (LENGTH_MEASURE( 1.000000000000000082E-05 ), #5433, 'distance_accuracy_value', 'NONE');
#14100=ORIENTED_EDGE ( 'NONE', *, *, #12286, .T. ) ;
#14116=ADVANCED_FACE ( 'NONE', ( #11862 ), #16839, .T. ) ;
#14186=DIRECTION ( 'NONE',  ( -0.8660254037844360431, -0.5000000000000046629, 0.000000000000000000 ) ) ;
#14188=( GEOMETRIC_REPRESENTATION_CONTEXT ( 3 ) GLOBAL_UNCERTAINTY_ASSIGNED_CONTEXT ( ( #14052 ) ) GLOBAL_UNIT_ASSIGNED_CONTEXT ( ( #5433, #10098, #18500 ) ) REPRESENTATION_CONTEXT ( 'NONE', 'WORKASPACE' ) );
#14192=ORIENTED_EDGE ( 'NONE', *, *, #20416, .T. ) ;
#14222=CARTESIAN_POINT ( 'NONE',  ( 58.37797649651341203, 276.8427481158987007, -28.99999999999998934 ) ) ;
#14247=VECTOR ( 'NONE', #1130, 1000.000000000000114 ) ;
#14266=ORIENTED_EDGE ( 'NONE', *, *, #14586, .T. ) ;
#14378=CARTESIAN_POINT ( 'NONE',  ( 85.37797649651368204, 230.0773763115391262, -0.9999999999999826805 ) ) ;
#14584=CARTESIAN_POINT ( 'NONE',  ( 57.15554463217811332, 244.9600622137188850, -13.99999999999998046 ) ) ;
#14586=EDGE_CURVE ( 'NONE', #16809, #15204, #20096, .T. ) ;
#14643=DIRECTION ( 'NONE',  ( -0.000000000000000000, -0.000000000000000000, -1.000000000000000000 ) ) ;
#14782=DIRECTION ( 'NONE',  ( -0.8660254037844348218, -0.5000000000000064393, 0.000000000000000000 ) ) ;
#14797=DIRECTION ( 'NONE',  ( 0.000000000000000000, -0.000000000000000000, 1.000000000000000000 ) ) ;
#14799=CARTESIAN_POINT ( 'NONE',  ( 57.15554463217811332, 244.9600622137188850, -13.99999999999998046 ) ) ;
#14825=LINE ( 'NONE', #6410, #2376 ) ;
#14937=EDGE_CURVE ( 'NONE', #19670, #1594, #20, .T. ) ;
#14939=CARTESIAN_POINT ( 'NONE',  ( 61.99529059433385925, 216.5773763115390125, -5.999999999999973355 ) ) ;
#15047=DIRECTION ( 'NONE',  ( 0.5000000000000041078, -0.8660254037844363761, 0.000000000000000000 ) ) ;
#15056=LINE ( 'NONE', #16830, #1214 ) ;
#15089=DIRECTION ( 'NONE',  ( -0.5000000000000045519, 0.8660254037844360431, 0.000000000000000000 ) ) ;
#15097=ORIENTED_EDGE ( 'NONE', *, *, #10637, .T. ) ;
#15151=LINE ( 'NONE', #3988, #18312 ) ;
#15199=VERTEX_POINT ( 'NONE', #15515 ) ;
#15204=VERTEX_POINT ( 'NONE', #4155 ) ;
#15228=VECTOR ( 'NONE', #14643, 1000.000000000000000 ) ;
#15262=DIRECTION ( 'NONE',  ( -0.5000000000000045519, 0.8660254037844360431, 0.000000000000000000 ) ) ;
#15288=ORIENTED_EDGE ( 'NONE', *, *, #5764, .F. ) ;
#15301=CARTESIAN_POINT ( 'NONE',  ( 34.99529059433362477, 263.3427481158986438, -28.99999999999998934 ) ) ;
#15314=APPLICATION_CONTEXT ( 'automotive_design' ) ;
#15325=CARTESIAN_POINT ( 'NONE',  ( 61.99529059433388767, 216.5773763115390693, -28.99999999999998934 ) ) ;
#15396=CARTESIAN_POINT ( 'NONE',  ( 58.37797649651341203, 276.8427481158987007, -0.9999999999999826805 ) ) ;
#15425=CARTESIAN_POINT ( 'NONE',  ( 34.99529059433359635, 263.3427481158985870, -22.00000000000000355 ) ) ;
#15459=ORIENTED_EDGE ( 'NONE', *, *, #20416, .F. ) ;
#15509=ORIENTED_EDGE ( 'NONE', *, *, #4882, .T. ) ;
#15515=CARTESIAN_POINT ( 'NONE',  ( 34.99529059433362477, 263.3427481158986438, -28.99999999999998934 ) ) ;
#15622=DIRECTION ( 'NONE',  ( 0.000000000000000000, 0.000000000000000000, -1.000000000000000000 ) ) ;
#15736=FACE_OUTER_BOUND ( 'NONE', #5811, .T. ) ;
#15781=DIRECTION ( 'NONE',  ( 0.7559289460184535070, 0.000000000000000000, -0.6546536707079781969 ) ) ;
#15791=ADVANCED_FACE ( 'NONE', ( #17904 ), #12925, .T. ) ;
#15817=EDGE_LOOP ( 'NONE', ( #18338, #19023, #15509, #17552 ) ) ;
#15867=CARTESIAN_POINT ( 'NONE',  ( 58.37797649651341203, 276.8427481158987007, -26.99999999999999289 ) ) ;
#15903=CARTESIAN_POINT ( 'NONE',  ( 0.000000000000000000, 0.000000000000000000, 0.000000000000000000 ) ) ;
#15959=DIRECTION ( 'NONE',  ( 0.5000000000000041078, -0.8660254037844363761, 0.000000000000000000 ) ) ;
#15991=FACE_OUTER_BOUND ( 'NONE', #5077, .T. ) ;
#16003=ORIENTED_EDGE ( 'NONE', *, *, #8125, .T. ) ;
#16131=ORIENTED_EDGE ( 'NONE', *, *, #11730, .F. ) ;
#16217=ORIENTED_EDGE ( 'NONE', *, *, #18216, .F. ) ;
#16242=AXIS2_PLACEMENT_3D ( 'NONE', #5667, #10226, #15047 ) ;
#16263=ORIENTED_EDGE ( 'NONE', *, *, #2110, .F. ) ;
#16334=AXIS2_PLACEMENT_3D ( 'NONE', #4215, #13869, #15781 ) ;
#16383=DIRECTION ( 'NONE',  ( 3.965082230804136136E-15, 7.930164461608272272E-15, 1.000000000000000000 ) ) ;
#16405=PLANE ( 'NONE',  #10155 ) ;
#16478=LINE ( 'NONE', #11815, #4787 ) ;
#16540=EDGE_CURVE ( 'NONE', #1594, #10851, #9838, .T. ) ;
#16559=ORIENTED_EDGE ( 'NONE', *, *, #5764, .T. ) ;
#16632=ORIENTED_EDGE ( 'NONE', *, *, #2566, .F. ) ;
#16727=ORIENTED_EDGE ( 'NONE', *, *, #8125, .F. ) ;
#16747=VECTOR ( 'NONE', #19738, 1000.000000000000114 ) ;
#16809=VERTEX_POINT ( 'NONE', #7396 ) ;
#16830=CARTESIAN_POINT ( 'NONE',  ( 85.37797649651368204, 230.0773763115391262, -0.9999999999999826805 ) ) ;
#16839=PLANE ( 'NONE',  #12064 ) ;
#16869=AXIS2_PLACEMENT_3D ( 'NONE', #18488, #2697, #3959 ) ;
#16914=DIRECTION ( 'NONE',  ( 0.000000000000000000, 0.000000000000000000, 1.000000000000000000 ) ) ;
#16967=AXIS2_PLACEMENT_3D ( 'NONE', #8111, #397, #6521 ) ;
#17022=ORIENTED_EDGE ( 'NONE', *, *, #20882, .T. ) ;
#17040=PRODUCT_DEFINITION_SHAPE ( 'NONE', 'NONE',  #12880 ) ;
#17060=APPLICATION_CONTEXT ( 'automotive_design' ) ;
#17131=EDGE_LOOP ( 'NONE', ( #12298, #214, #4642, #14192 ) ) ;
#17239=EDGE_CURVE ( 'NONE', #2539, #10247, #3889, .T. ) ;
#17271=ORIENTED_EDGE ( 'NONE', *, *, #12286, .F. ) ;
#17303=CARTESIAN_POINT ( 'NONE',  ( 57.15554463217811332, 244.9600622137188850, -13.99999999999998046 ) ) ;
#17310=AXIS2_PLACEMENT_3D ( 'NONE', #4677, #3194, #2995 ) ;
#17343=MECHANICAL_DESIGN_GEOMETRIC_PRESENTATION_REPRESENTATION('',(#11923),#1094);
#17375=VERTEX_POINT ( 'NONE', #5026 ) ;
#17521=PLANE ( 'NONE',  #2503 ) ;
#17535=( LENGTH_UNIT ( ) NAMED_UNIT ( * ) SI_UNIT ( .MILLI., .METRE. ) );
#17540=ORIENTED_EDGE ( 'NONE', *, *, #9117, .F. ) ;
#17552=ORIENTED_EDGE ( 'NONE', *, *, #1106, .T. ) ;
#17637=VERTEX_POINT ( 'NONE', #14378 ) ;
#17717=EDGE_CURVE ( 'NONE', #2773, #15199, #4476, .T. ) ;
#17764=CARTESIAN_POINT ( 'NONE',  ( 58.37797649651341203, 276.8427481158987007, -28.99999999999998934 ) ) ;
#17821=CARTESIAN_POINT ( 'NONE',  ( 59.39721438298058587, 215.0773763115390125, -22.00000000000000355 ) ) ;
#17833=VECTOR ( 'NONE', #18725, 1000.000000000000114 ) ;
#17849=( NAMED_UNIT ( * ) SI_UNIT ( $, .STERADIAN. ) SOLID_ANGLE_UNIT ( ) );
#17865=ORIENTED_EDGE ( 'NONE', *, *, #968, .F. ) ;
#17898=CARTESIAN_POINT ( 'NONE',  ( -78.28193223680408153, 135.5882839488078844, -1.028642961561239307E-12 ) ) ;
#17903=CARTESIAN_POINT ( 'NONE',  ( 59.39721438298058587, 215.0773763115390125, -22.00000000000000355 ) ) ;
#17904=FACE_OUTER_BOUND ( 'NONE', #1915, .T. ) ;
#17917=ADVANCED_FACE ( 'NONE', ( #5638 ), #5538, .T. ) ;
#17983=VECTOR ( 'NONE', #19268, 1000.000000000000114 ) ;
#17992=AXIS2_PLACEMENT_3D ( 'NONE', #5778, #14186, #12479 ) ;
#18043=AXIS2_PLACEMENT_3D ( 'NONE', #5683, #8880, #5370 ) ;
#18216=EDGE_CURVE ( 'NONE', #18774, #4855, #983, .T. ) ;
#18233=AXIS2_PLACEMENT_3D ( 'NONE', #15903, #1274, #19656 ) ;
#18262=LINE ( 'NONE', #3728, #16747 ) ;
#18312=VECTOR ( 'NONE', #5452, 1000.000000000000000 ) ;
#18338=ORIENTED_EDGE ( 'NONE', *, *, #20482, .F. ) ;
#18387=ORIENTED_EDGE ( 'NONE', *, *, #18216, .T. ) ;
#18422=ORIENTED_EDGE ( 'NONE', *, *, #18738, .F. ) ;
#18447=CARTESIAN_POINT ( 'NONE',  ( 54.65554463217808490, 249.2901892326410689, -13.99999999999998046 ) ) ;
#18451=DIRECTION ( 'NONE',  ( 0.8660254037844370423, 0.5000000000000027756, 0.000000000000000000 ) ) ;
#18488=CARTESIAN_POINT ( 'NONE',  ( -105.2819322368043515, 182.3536557531674873, -1.028642961561239307E-12 ) ) ;
#18500=( NAMED_UNIT ( * ) SI_UNIT ( $, .STERADIAN. ) SOLID_ANGLE_UNIT ( ) );
#18512=CARTESIAN_POINT ( 'NONE',  ( 34.99529059433362477, 263.3427481158986438, -28.99999999999998934 ) ) ;
#18551=ORIENTED_EDGE ( 'NONE', *, *, #3433, .T. ) ;
#18582=EDGE_CURVE ( 'NONE', #4855, #7191, #19920, .T. ) ;
#18616=EDGE_LOOP ( 'NONE', ( #20598, #16217, #14100, #6655 ) ) ;
#18675=ORIENTED_EDGE ( 'NONE', *, *, #7070, .T. ) ;
#18685=CARTESIAN_POINT ( 'NONE',  ( 61.99529059433388767, 216.5773763115390693, -28.99999999999998934 ) ) ;
#18697=CARTESIAN_POINT ( 'NONE',  ( 85.37797649651368204, 230.0773763115391262, -26.99999999999999289 ) ) ;
#18725=DIRECTION ( 'NONE',  ( -0.5000000000000045519, 0.8660254037844360431, 0.000000000000000000 ) ) ;
#18738=EDGE_CURVE ( 'NONE', #10851, #2949, #9301, .T. ) ;
#18774=VERTEX_POINT ( 'NONE', #19385 ) ;
#18885=ORIENTED_EDGE ( 'NONE', *, *, #8734, .F. ) ;
#18948=ADVANCED_FACE ( 'NONE', ( #10129 ), #19578, .T. ) ;
#18964=VERTEX_POINT ( 'NONE', #10238 ) ;
#18972=CARTESIAN_POINT ( 'NONE',  ( 47.11964624731579221, 270.3427481158987007, -13.99999999999998757 ) ) ;
#18978=LINE ( 'NONE', #15301, #5168 ) ;
#19023=ORIENTED_EDGE ( 'NONE', *, *, #17239, .F. ) ;
#19041=VERTEX_POINT ( 'NONE', #20211 ) ;
#19053=ORIENTED_EDGE ( 'NONE', *, *, #13844, .F. ) ;
#19080=CARTESIAN_POINT ( 'NONE',  ( 59.39721438298058587, 215.0773763115390125, -5.999999999999973355 ) ) ;
#19158=VECTOR ( 'NONE', #18451, 1000.000000000000114 ) ;
#19245=CARTESIAN_POINT ( 'NONE',  ( 59.39721438298058587, 215.0773763115390125, -22.00000000000000355 ) ) ;
#19268=DIRECTION ( 'NONE',  ( -0.5000000000000045519, 0.8660254037844360431, 0.000000000000000000 ) ) ;
#19361=VECTOR ( 'NONE', #1738, 1000.000000000000000 ) ;
#19385=CARTESIAN_POINT ( 'NONE',  ( 59.65554463217813463, 240.6299351947967011, -13.99999999999998046 ) ) ;
#19424=( NAMED_UNIT ( * ) PLANE_ANGLE_UNIT ( ) SI_UNIT ( $, .RADIAN. ) );
#19525=ORIENTED_EDGE ( 'NONE', *, *, #91, .F. ) ;
#19578=PLANE ( 'NONE',  #10448 ) ;
#19584=DIRECTION ( 'NONE',  ( -0.8660254037844361541, -0.5000000000000044409, 5.976026924694052093E-17 ) ) ;
#19620=ORIENTED_EDGE ( 'NONE', *, *, #14586, .F. ) ;
#19656=DIRECTION ( 'NONE',  ( 1.000000000000000000, 0.000000000000000000, 0.000000000000000000 ) ) ;
#19670=VERTEX_POINT ( 'NONE', #2343 ) ;
#19738=DIRECTION ( 'NONE',  ( -0.5000000000000045519, 0.8660254037844360431, 0.000000000000000000 ) ) ;
#19765=EDGE_CURVE ( 'NONE', #1958, #16809, #20038, .T. ) ;
#19904=VECTOR ( 'NONE', #12311, 1000.000000000000227 ) ;
#19920=LINE ( 'NONE', #18447, #12505 ) ;
#19993=AXIS2_PLACEMENT_3D ( 'NONE', #14939, #5566, #12059 ) ;
#20026=CARTESIAN_POINT ( 'NONE',  ( 34.99529059433359635, 263.3427481158985870, -5.999999999999973355 ) ) ;
#20038=LINE ( 'NONE', #3605, #19158 ) ;
#20068=DIRECTION ( 'NONE',  ( -1.000000000000000000, 0.000000000000000000, -0.000000000000000000 ) ) ;
#20096=LINE ( 'NONE', #20299, #17833 ) ;
#20198=EDGE_LOOP ( 'NONE', ( #7913, #19053, #16632, #2776, #16131, #3316, #5171, #18885, #19525, #7887, #8826 ) ) ;
#20211=CARTESIAN_POINT ( 'NONE',  ( 59.39721438298058587, 215.0773763115390125, -22.00000000000000355 ) ) ;
#20296=ADVANCED_FACE ( 'NONE', ( #11178 ), #4814, .F. ) ;
#20299=CARTESIAN_POINT ( 'NONE',  ( 85.37797649651368204, 230.0773763115391262, 1.000000000000017097 ) ) ;
#20391=PRODUCT_DEFINITION_CONTEXT ( 'detailed design', #17060, 'design' ) ;
#20400=ORIENTED_EDGE ( 'NONE', *, *, #19765, .T. ) ;
#20416=EDGE_CURVE ( 'NONE', #1588, #2098, #8291, .T. ) ;
#20459=EDGE_LOOP ( 'NONE', ( #10959, #16559, #3124, #17022, #10864, #13317, #16003, #1643, #20715, #6712, #9739 ) ) ;
#20462=EDGE_LOOP ( 'NONE', ( #20612, #15459, #3547, #11544 ) ) ;
#20482=EDGE_CURVE ( 'NONE', #10247, #17375, #10294, .T. ) ;
#20590=ORIENTED_EDGE ( 'NONE', *, *, #9117, .T. ) ;
#20591=ORIENTED_EDGE ( 'NONE', *, *, #20882, .F. ) ;
#20598=ORIENTED_EDGE ( 'NONE', *, *, #18582, .F. ) ;
#20612=ORIENTED_EDGE ( 'NONE', *, *, #5564, .F. ) ;
#20630=DIRECTION ( 'NONE',  ( -0.5000000000000045519, 0.8660254037844360431, 0.000000000000000000 ) ) ;
#20646=VECTOR ( 'NONE', #20630, 1000.000000000000114 ) ;
#20715=ORIENTED_EDGE ( 'NONE', *, *, #20482, .T. ) ;
#20784=PLANE ( 'NONE',  #17310 ) ;
#20807=CARTESIAN_POINT ( 'NONE',  ( 61.99529059433388767, 216.5773763115390693, 1.000000000000017097 ) ) ;
#20882=EDGE_CURVE ( 'NONE', #2259, #1594, #10366, .T. ) ;
#20968=COLOUR_RGB('Light Blue',0.38,0.62,0.78);
#20969=FILL_AREA_STYLE_COLOUR('',#20968);
#20970=FILL_AREA_STYLE('',(#20969));
#20971=SURFACE_STYLE_FILL_AREA(#20970);
#20972=SURFACE_SIDE_STYLE('',(#20971));
#20973=SURFACE_STYLE_USAGE(.BOTH.,#20972);
#20974=PRESENTATION_STYLE_ASSIGNMENT((#20973));
ENDSEC;
END-ISO-10303-21;
